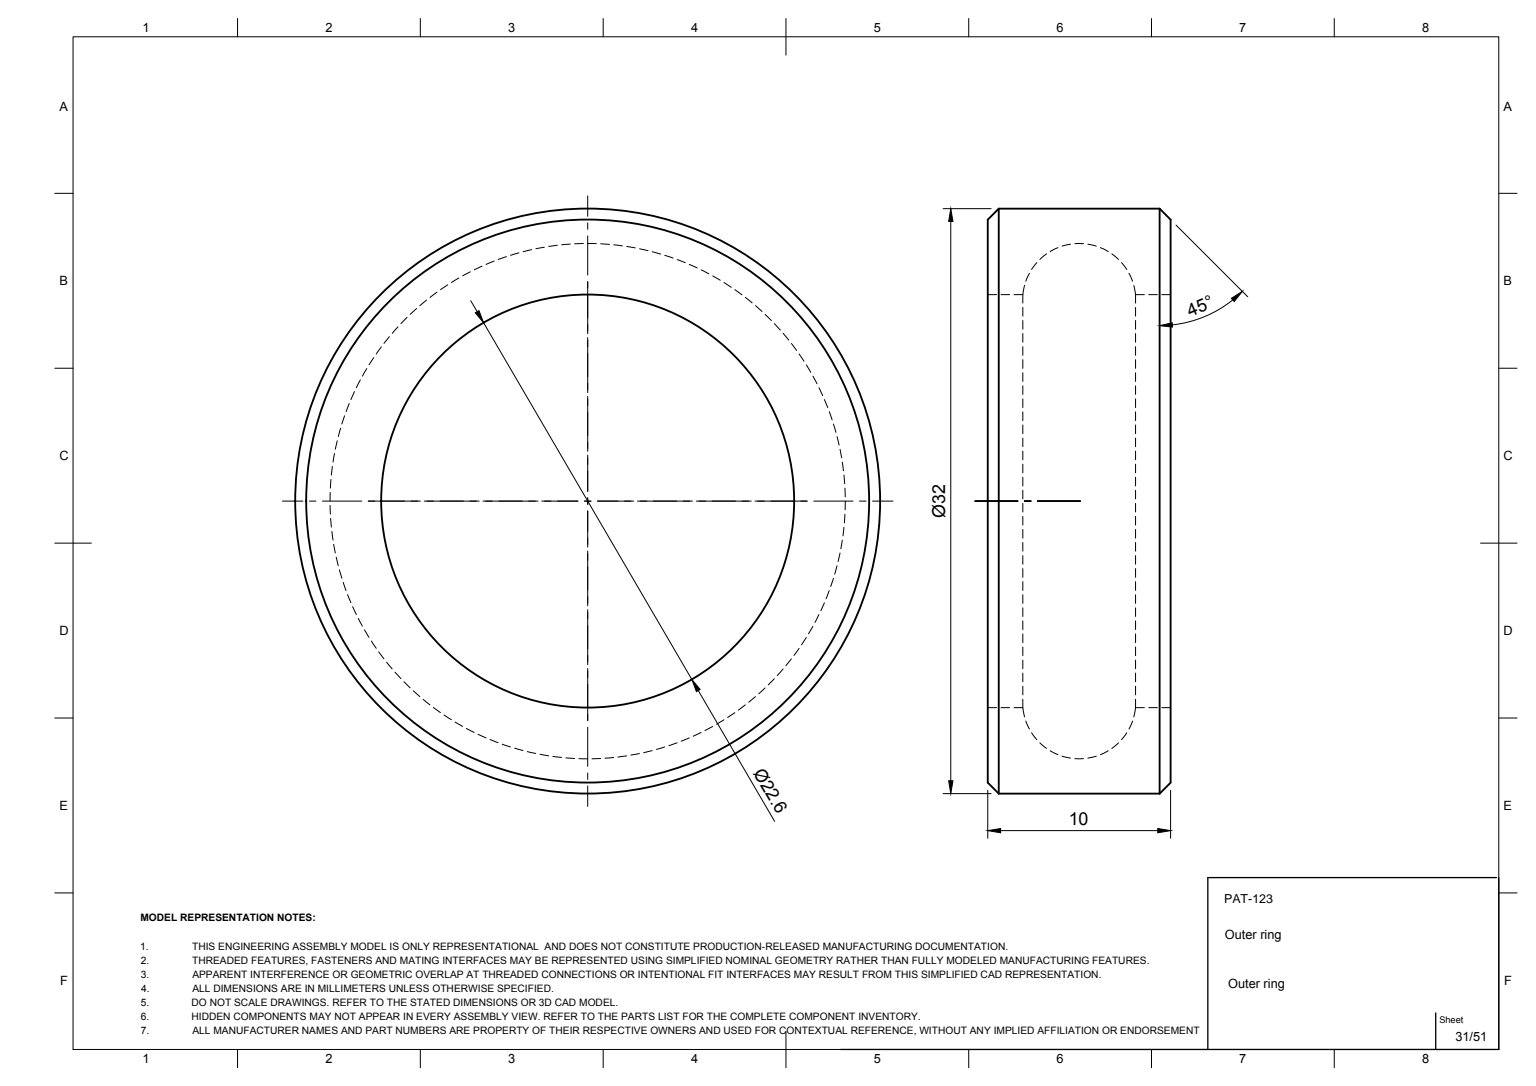
ISO-10303-21;
HEADER;
/* Generated by software containing ST-Developer
 * from STEP Tools, Inc. (www.steptools.com) 
 */

FILE_DESCRIPTION(
/* description */ ('Worm-less right-angle friction wheel drive'),
/* implementation_level */ '2;1');

FILE_NAME(
/* name */ 'Outer ring.step',
/* time_stamp */ '2026-10-28T03:22:36-07:00',
/* author */ (''),
/* organization */ (''),
/* preprocessor_version */ 'ST-DEVELOPER v20.2',
/* originating_system */ 'Autodesk Translation Framework v15.17.0.0',
/* authorisation */ '');

FILE_SCHEMA (('AUTOMOTIVE_DESIGN { 1 0 10303 214 3 1 1 }'));
ENDSEC;

DATA;
#10=MECHANICAL_DESIGN_GEOMETRIC_PRESENTATION_REPRESENTATION('',(#636),#17046);
#450=TOROIDAL_SURFACE('',#9283,1.1,0.309556);
#461=CONICAL_SURFACE('',#9294,1.57,0.785398163397449);
#462=CONICAL_SURFACE('',#9298,1.57,0.785398163397449);
#542=SHAPE_REPRESENTATION_RELATIONSHIP('SRR','None',#17286,#589);
#589=ADVANCED_BREP_SHAPE_REPRESENTATION('',(#689),#17022);
#636=STYLED_ITEM('',(#17591),#689);
#689=MANIFOLD_SOLID_BREP('Body1',#8192);
#908=FACE_BOUND('',#2129,.T.);
#909=FACE_BOUND('',#2134,.T.);
#1081=PLANE('',#9291);
#1082=PLANE('',#9300);
#1467=FACE_OUTER_BOUND('',#2126,.T.);
#1468=FACE_OUTER_BOUND('',#2127,.T.);
#1469=FACE_OUTER_BOUND('',#2128,.T.);
#1470=FACE_OUTER_BOUND('',#2130,.T.);
#1471=FACE_OUTER_BOUND('',#2131,.T.);
#1472=FACE_OUTER_BOUND('',#2132,.T.);
#1473=FACE_OUTER_BOUND('',#2133,.T.);
#1474=FACE_OUTER_BOUND('',#2135,.T.);
#2126=EDGE_LOOP('',(#6698,#6699,#6700,#6701,#6702,#6703));
#2127=EDGE_LOOP('',(#6704,#6705,#6706,#6707,#6708));
#2128=EDGE_LOOP('',(#6709));
#2129=EDGE_LOOP('',(#6710));
#2130=EDGE_LOOP('',(#6711,#6712,#6713,#6714));
#2131=EDGE_LOOP('',(#6715,#6716,#6717,#6718));
#2132=EDGE_LOOP('',(#6719,#6720,#6721,#6722));
#2133=EDGE_LOOP('',(#6723));
#2134=EDGE_LOOP('',(#6724));
#2135=EDGE_LOOP('',(#6725,#6726,#6727,#6728,#6729));
#2702=LINE('',#15444,#3242);
#2703=LINE('',#15453,#3243);
#2704=LINE('',#15457,#3244);
#2705=LINE('',#15461,#3245);
#2706=LINE('',#15464,#3246);
#3242=VECTOR('',#11196,1.129765);
#3243=VECTOR('',#11207,1.57);
#3244=VECTOR('',#11212,1.6);
#3245=VECTOR('',#11217,1.57);
#3246=VECTOR('',#11222,1.129765);
#3712=CIRCLE('',#9284,1.129765);
#3713=CIRCLE('',#9285,1.129765);
#3714=CIRCLE('',#9286,0.309556);
#3715=CIRCLE('',#9287,1.129765);
#3716=CIRCLE('',#9288,1.129765);
#3717=CIRCLE('',#9290,1.129765);
#3718=CIRCLE('',#9292,1.54);
#3719=CIRCLE('',#9293,1.129765);
#3720=CIRCLE('',#9295,1.6);
#3721=CIRCLE('',#9297,1.6);
#3722=CIRCLE('',#9299,1.54);
#4255=VERTEX_POINT('',#15432);
#4256=VERTEX_POINT('',#15433);
#4257=VERTEX_POINT('',#15436);
#4258=VERTEX_POINT('',#15438);
#4259=VERTEX_POINT('',#15442);
#4260=VERTEX_POINT('',#15446);
#4261=VERTEX_POINT('',#15448);
#4262=VERTEX_POINT('',#15451);
#4263=VERTEX_POINT('',#15455);
#4264=VERTEX_POINT('',#15459);
#5118=EDGE_CURVE('',#4255,#4256,#3712,.T.);
#5119=EDGE_CURVE('',#4256,#4255,#3713,.T.);
#5120=EDGE_CURVE('',#4256,#4257,#3714,.T.);
#5121=EDGE_CURVE('',#4258,#4257,#3715,.T.);
#5122=EDGE_CURVE('',#4257,#4258,#3716,.T.);
#5123=EDGE_CURVE('',#4259,#4259,#3717,.T.);
#5124=EDGE_CURVE('',#4259,#4258,#2702,.T.);
#5125=EDGE_CURVE('',#4260,#4260,#3718,.T.);
#5126=EDGE_CURVE('',#4261,#4261,#3719,.T.);
#5127=EDGE_CURVE('',#4262,#4262,#3720,.T.);
#5128=EDGE_CURVE('',#4262,#4260,#2703,.T.);
#5129=EDGE_CURVE('',#4263,#4263,#3721,.T.);
#5130=EDGE_CURVE('',#4263,#4262,#2704,.T.);
#5131=EDGE_CURVE('',#4264,#4264,#3722,.T.);
#5132=EDGE_CURVE('',#4264,#4263,#2705,.T.);
#5133=EDGE_CURVE('',#4255,#4261,#2706,.T.);
#6698=ORIENTED_EDGE('',*,*,#5118,.F.);
#6699=ORIENTED_EDGE('',*,*,#5119,.F.);
#6700=ORIENTED_EDGE('',*,*,#5120,.T.);
#6701=ORIENTED_EDGE('',*,*,#5121,.F.);
#6702=ORIENTED_EDGE('',*,*,#5122,.F.);
#6703=ORIENTED_EDGE('',*,*,#5120,.F.);
#6704=ORIENTED_EDGE('',*,*,#5123,.T.);
#6705=ORIENTED_EDGE('',*,*,#5124,.T.);
#6706=ORIENTED_EDGE('',*,*,#5121,.T.);
#6707=ORIENTED_EDGE('',*,*,#5122,.T.);
#6708=ORIENTED_EDGE('',*,*,#5124,.F.);
#6709=ORIENTED_EDGE('',*,*,#5125,.F.);
#6710=ORIENTED_EDGE('',*,*,#5126,.T.);
#6711=ORIENTED_EDGE('',*,*,#5127,.F.);
#6712=ORIENTED_EDGE('',*,*,#5128,.T.);
#6713=ORIENTED_EDGE('',*,*,#5125,.T.);
#6714=ORIENTED_EDGE('',*,*,#5128,.F.);
#6715=ORIENTED_EDGE('',*,*,#5129,.F.);
#6716=ORIENTED_EDGE('',*,*,#5130,.T.);
#6717=ORIENTED_EDGE('',*,*,#5127,.T.);
#6718=ORIENTED_EDGE('',*,*,#5130,.F.);
#6719=ORIENTED_EDGE('',*,*,#5131,.F.);
#6720=ORIENTED_EDGE('',*,*,#5132,.T.);
#6721=ORIENTED_EDGE('',*,*,#5129,.T.);
#6722=ORIENTED_EDGE('',*,*,#5132,.F.);
#6723=ORIENTED_EDGE('',*,*,#5131,.T.);
#6724=ORIENTED_EDGE('',*,*,#5123,.F.);
#6725=ORIENTED_EDGE('',*,*,#5118,.T.);
#6726=ORIENTED_EDGE('',*,*,#5119,.T.);
#6727=ORIENTED_EDGE('',*,*,#5133,.T.);
#6728=ORIENTED_EDGE('',*,*,#5126,.F.);
#6729=ORIENTED_EDGE('',*,*,#5133,.F.);
#7651=CYLINDRICAL_SURFACE('',#9289,1.129765);
#7652=CYLINDRICAL_SURFACE('',#9296,1.6);
#7653=CYLINDRICAL_SURFACE('',#9301,1.129765);
#7959=ADVANCED_FACE('',(#1467),#450,.F.);
#7960=ADVANCED_FACE('',(#1468),#7651,.F.);
#7961=ADVANCED_FACE('',(#1469,#908),#1081,.T.);
#7962=ADVANCED_FACE('',(#1470),#461,.T.);
#7963=ADVANCED_FACE('',(#1471),#7652,.T.);
#7964=ADVANCED_FACE('',(#1472),#462,.T.);
#7965=ADVANCED_FACE('',(#1473,#909),#1082,.T.);
#7966=ADVANCED_FACE('',(#1474),#7653,.F.);
#8192=CLOSED_SHELL('',(#7959,#7960,#7961,#7962,#7963,#7964,#7965,#7966));
#9282=AXIS2_PLACEMENT_3D('',#15430,#11178,#11179);
#9283=AXIS2_PLACEMENT_3D('',#15431,#11180,#11181);
#9284=AXIS2_PLACEMENT_3D('',#15434,#11182,#11183);
#9285=AXIS2_PLACEMENT_3D('',#15435,#11184,#11185);
#9286=AXIS2_PLACEMENT_3D('',#15437,#11186,#11187);
#9287=AXIS2_PLACEMENT_3D('',#15439,#11188,#11189);
#9288=AXIS2_PLACEMENT_3D('',#15440,#11190,#11191);
#9289=AXIS2_PLACEMENT_3D('',#15441,#11192,#11193);
#9290=AXIS2_PLACEMENT_3D('',#15443,#11194,#11195);
#9291=AXIS2_PLACEMENT_3D('',#15445,#11197,#11198);
#9292=AXIS2_PLACEMENT_3D('',#15447,#11199,#11200);
#9293=AXIS2_PLACEMENT_3D('',#15449,#11201,#11202);
#9294=AXIS2_PLACEMENT_3D('',#15450,#11203,#11204);
#9295=AXIS2_PLACEMENT_3D('',#15452,#11205,#11206);
#9296=AXIS2_PLACEMENT_3D('',#15454,#11208,#11209);
#9297=AXIS2_PLACEMENT_3D('',#15456,#11210,#11211);
#9298=AXIS2_PLACEMENT_3D('',#15458,#11213,#11214);
#9299=AXIS2_PLACEMENT_3D('',#15460,#11215,#11216);
#9300=AXIS2_PLACEMENT_3D('',#15462,#11218,#11219);
#9301=AXIS2_PLACEMENT_3D('',#15463,#11220,#11221);
#11178=DIRECTION('axis',(0.,0.,1.));
#11179=DIRECTION('refdir',(1.,0.,0.));
#11180=DIRECTION('center_axis',(0.,-1.,0.));
#11181=DIRECTION('ref_axis',(0.,0.,-1.));
#11182=DIRECTION('center_axis',(0.,-1.,0.));
#11183=DIRECTION('ref_axis',(1.,0.,0.));
#11184=DIRECTION('center_axis',(0.,-1.,0.));
#11185=DIRECTION('ref_axis',(1.,0.,0.));
#11186=DIRECTION('center_axis',(1.,0.,1.22464679914735E-16));
#11187=DIRECTION('ref_axis',(-1.22464679914735E-16,0.,1.));
#11188=DIRECTION('center_axis',(0.,1.,0.));
#11189=DIRECTION('ref_axis',(1.,0.,0.));
#11190=DIRECTION('center_axis',(0.,1.,0.));
#11191=DIRECTION('ref_axis',(1.,0.,0.));
#11192=DIRECTION('center_axis',(0.,-1.,0.));
#11193=DIRECTION('ref_axis',(1.,0.,0.));
#11194=DIRECTION('center_axis',(0.,-1.,0.));
#11195=DIRECTION('ref_axis',(1.,0.,0.));
#11196=DIRECTION('',(0.,1.,0.));
#11197=DIRECTION('center_axis',(0.,1.,0.));
#11198=DIRECTION('ref_axis',(0.,0.,1.));
#11199=DIRECTION('center_axis',(0.,-1.,0.));
#11200=DIRECTION('ref_axis',(1.,0.,0.));
#11201=DIRECTION('center_axis',(0.,-1.,0.));
#11202=DIRECTION('ref_axis',(1.,0.,0.));
#11203=DIRECTION('center_axis',(0.,-1.,0.));
#11204=DIRECTION('ref_axis',(1.,0.,0.));
#11205=DIRECTION('center_axis',(0.,-1.,0.));
#11206=DIRECTION('ref_axis',(1.,0.,0.));
#11207=DIRECTION('',(0.707106781186548,0.707106781186547,8.65956056235494E-17));
#11208=DIRECTION('center_axis',(0.,-1.,0.));
#11209=DIRECTION('ref_axis',(1.,0.,0.));
#11210=DIRECTION('center_axis',(0.,-1.,0.));
#11211=DIRECTION('ref_axis',(1.,0.,0.));
#11212=DIRECTION('',(0.,1.,0.));
#11213=DIRECTION('center_axis',(0.,1.,0.));
#11214=DIRECTION('ref_axis',(1.,0.,0.));
#11215=DIRECTION('center_axis',(0.,-1.,0.));
#11216=DIRECTION('ref_axis',(1.,0.,0.));
#11217=DIRECTION('',(-0.707106781186548,0.707106781186547,-8.65956056235494E-17));
#11218=DIRECTION('center_axis',(0.,-1.,0.));
#11219=DIRECTION('ref_axis',(0.,0.,-1.));
#11220=DIRECTION('center_axis',(0.,-1.,0.));
#11221=DIRECTION('ref_axis',(1.,0.,0.));
#11222=DIRECTION('',(0.,1.,0.));
#15430=CARTESIAN_POINT('',(0.,0.,0.));
#15431=CARTESIAN_POINT('Origin',(0.,0.,0.));
#15432=CARTESIAN_POINT('',(-1.129765,0.308121667383195,-1.38356309103871E-16));
#15433=CARTESIAN_POINT('',(-1.38356309103871E-16,0.308121667383195,1.129765));
#15434=CARTESIAN_POINT('Origin',(0.,0.308121667383195,0.));
#15435=CARTESIAN_POINT('Origin',(0.,0.308121667383195,0.));
#15436=CARTESIAN_POINT('',(-1.38356309103871E-16,-0.308121667383195,1.129765));
#15437=CARTESIAN_POINT('Origin',(-1.34711147906209E-16,0.,1.1));
#15438=CARTESIAN_POINT('',(-1.129765,-0.308121667383195,1.38356309103871E-16));
#15439=CARTESIAN_POINT('Origin',(0.,-0.308121667383195,0.));
#15440=CARTESIAN_POINT('Origin',(0.,-0.308121667383195,0.));
#15441=CARTESIAN_POINT('Origin',(0.,0.,0.));
#15442=CARTESIAN_POINT('',(-1.129765,-0.5,-1.38356309103871E-16));
#15443=CARTESIAN_POINT('Origin',(0.,-0.5,0.));
#15444=CARTESIAN_POINT('',(-1.129765,0.,-1.38356309103871E-16));
#15445=CARTESIAN_POINT('Origin',(1.54,0.5,0.));
#15446=CARTESIAN_POINT('',(-1.54,0.5,-1.88595607068692E-16));
#15447=CARTESIAN_POINT('Origin',(0.,0.5,0.));
#15448=CARTESIAN_POINT('',(-1.129765,0.5,-1.38356309103871E-16));
#15449=CARTESIAN_POINT('Origin',(0.,0.5,0.));
#15450=CARTESIAN_POINT('Origin',(0.,0.47,0.));
#15451=CARTESIAN_POINT('',(-1.6,0.44,-1.95943487863577E-16));
#15452=CARTESIAN_POINT('Origin',(0.,0.44,0.));
#15453=CARTESIAN_POINT('',(-1.57,0.47,-1.92269547466134E-16));
#15454=CARTESIAN_POINT('Origin',(0.,0.,0.));
#15455=CARTESIAN_POINT('',(-1.6,-0.44,-1.95943487863577E-16));
#15456=CARTESIAN_POINT('Origin',(0.,-0.44,0.));
#15457=CARTESIAN_POINT('',(-1.6,0.,-1.95943487863577E-16));
#15458=CARTESIAN_POINT('Origin',(0.,-0.47,0.));
#15459=CARTESIAN_POINT('',(-1.54,-0.5,-1.88595607068692E-16));
#15460=CARTESIAN_POINT('Origin',(0.,-0.5,0.));
#15461=CARTESIAN_POINT('',(-1.57,-0.47,-1.92269547466134E-16));
#15462=CARTESIAN_POINT('Origin',(1.129765,-0.5,0.));
#15463=CARTESIAN_POINT('Origin',(0.,0.,0.));
#15464=CARTESIAN_POINT('',(-1.129765,0.,-1.38356309103871E-16));
#16969=UNCERTAINTY_MEASURE_WITH_UNIT(LENGTH_MEASURE(0.001),#17047,
'DISTANCE_ACCURACY_VALUE',
'Maximum model space distance between geometric entities at asserted c
onnectivities');
#16993=UNCERTAINTY_MEASURE_WITH_UNIT(LENGTH_MEASURE(0.001),#17047,
'DISTANCE_ACCURACY_VALUE',
'Maximum model space distance between geometric entities at asserted c
onnectivities');
#17022=(
GEOMETRIC_REPRESENTATION_CONTEXT(3)
GLOBAL_UNCERTAINTY_ASSIGNED_CONTEXT((#16969))
GLOBAL_UNIT_ASSIGNED_CONTEXT((#17047,#17049,#17050))
REPRESENTATION_CONTEXT('','3D')
);
#17046=(
GEOMETRIC_REPRESENTATION_CONTEXT(3)
GLOBAL_UNCERTAINTY_ASSIGNED_CONTEXT((#16993))
GLOBAL_UNIT_ASSIGNED_CONTEXT((#17047,#17049,#17050))
REPRESENTATION_CONTEXT('','3D')
);
#17047=(
LENGTH_UNIT()
NAMED_UNIT(*)
SI_UNIT(.CENTI.,.METRE.)
);
#17049=(
NAMED_UNIT(*)
PLANE_ANGLE_UNIT()
SI_UNIT($,.RADIAN.)
);
#17050=(
NAMED_UNIT(*)
SI_UNIT($,.STERADIAN.)
SOLID_ANGLE_UNIT()
);
#17079=SHAPE_DEFINITION_REPRESENTATION(#17131,#17286);
#17131=PRODUCT_DEFINITION_SHAPE('',$,#17339);
#17286=SHAPE_REPRESENTATION('',(#9282),#17022);
#17310=PRODUCT_DEFINITION_CONTEXT('part definition',#17468,'design');
#17339=PRODUCT_DEFINITION('Outer ring','Outer ring',#17391,#17310);
#17391=PRODUCT_DEFINITION_FORMATION('',$,#17498);
#17468=APPLICATION_CONTEXT(
'Core Data for Automotive Mechanical Design Process');
#17469=PRODUCT_CONTEXT('part definition',#17468,'mechanical');
#17498=PRODUCT('Outer ring','Outer ring','Outer ring',(#17469));
#17585=COLOUR_RGB('Grey',0.48,0.52,0.57);
#17586=FILL_AREA_STYLE_COLOUR('',#17585);
#17587=FILL_AREA_STYLE('',(#17586));
#17588=SURFACE_STYLE_FILL_AREA(#17587);
#17589=SURFACE_SIDE_STYLE('',(#17588));
#17590=SURFACE_STYLE_USAGE(.BOTH.,#17589);
#17591=PRESENTATION_STYLE_ASSIGNMENT((#17590));
ENDSEC;
END-ISO-10303-21;
